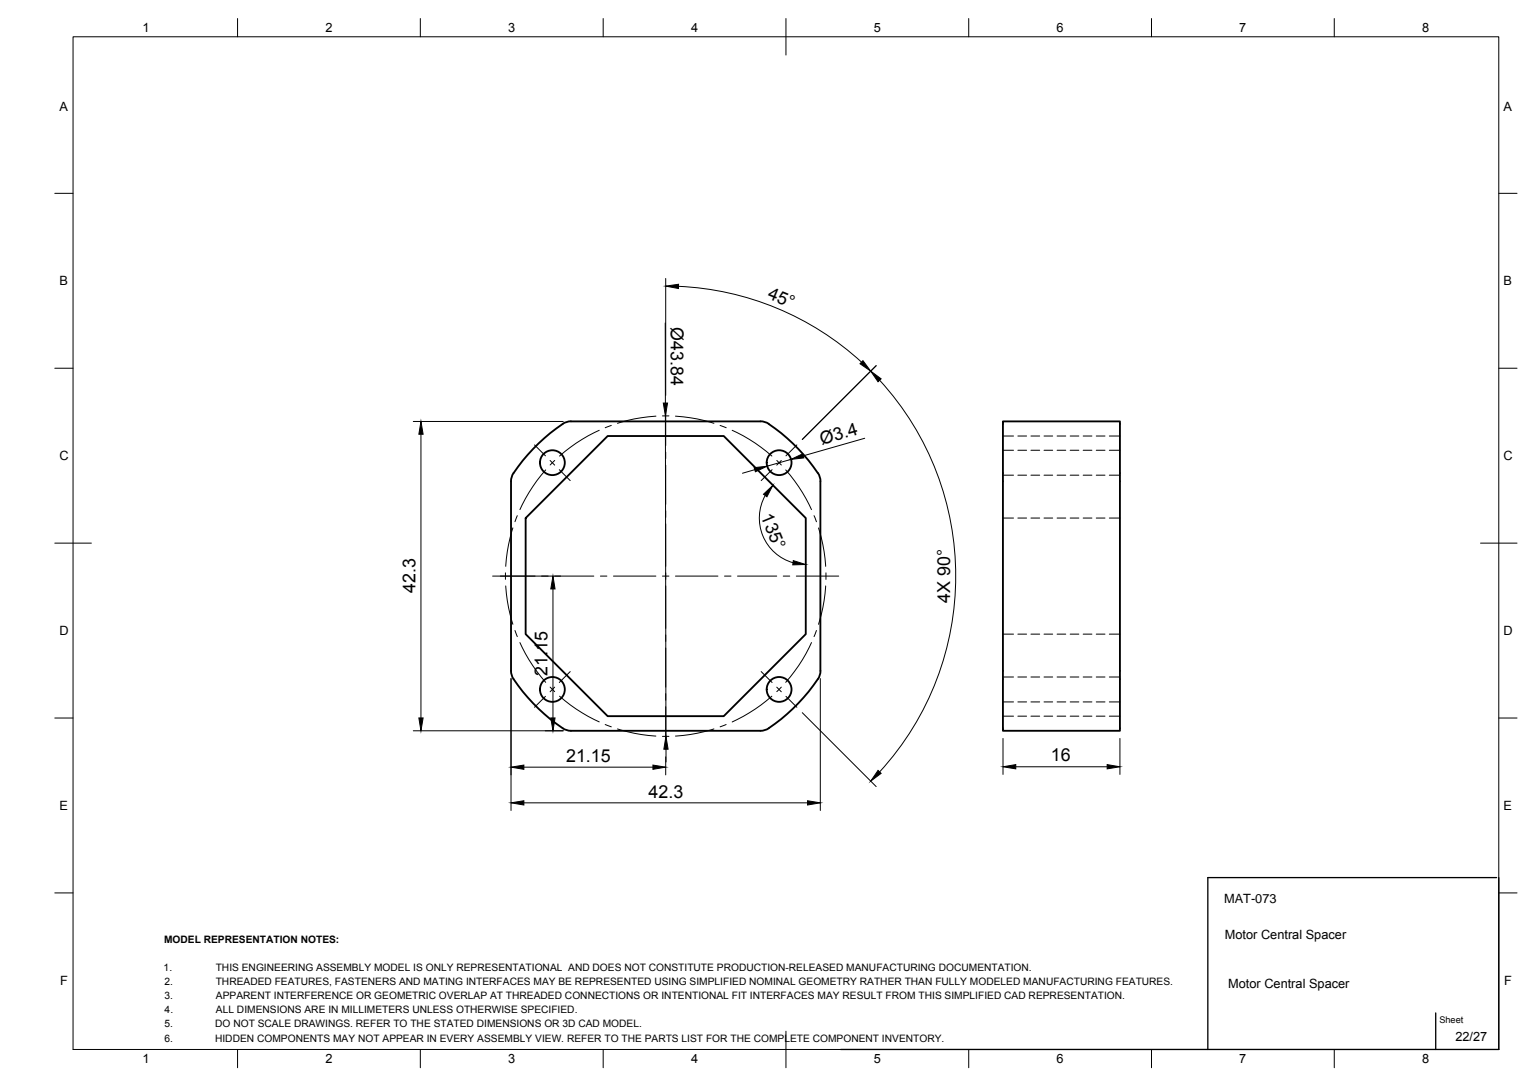
ISO-10303-21;
HEADER;
/* Generated by software containing ST-Developer
 * from STEP Tools, Inc. (www.steptools.com) 
 */

FILE_DESCRIPTION(
/* description */ ('CAx-IF Rec.Pracs.---Representation and Presentation of Product Manufa
cturing Information (PMI)---4.0---2014-10-13'),
/* implementation_level */ '2;1');

FILE_NAME(
/* name */ 'Motor Central Spacer.step',
/* time_stamp */ '2026-10-24T18:52:33-07:00',
/* author */ (''),
/* organization */ (''),
/* preprocessor_version */ 'ST-DEVELOPER v20.2',
/* originating_system */ 'Autodesk Translation Framework v15.17.0.0',
/* authorisation */ '');

FILE_SCHEMA (('AP242_MANAGED_MODEL_BASED_3D_ENGINEERING_MIM_LF { 1 0 10303 442 2 1 4 }'));
ENDSEC;

DATA;
#10=MECHANICAL_DESIGN_GEOMETRIC_PRESENTATION_REPRESENTATION('',(#438),#34876);
#372=SHAPE_REPRESENTATION_RELATIONSHIP('SRR','None',#35009,#405);
#405=ADVANCED_BREP_SHAPE_REPRESENTATION('',(#471),#34867);
#438=STYLED_ITEM('',(#35166),#471);
#471=MANIFOLD_SOLID_BREP('Motor Central Spacer',#19578);
#562=FACE_BOUND('',#6740,.T.);
#563=FACE_BOUND('',#6741,.T.);
#564=FACE_BOUND('',#6742,.T.);
#565=FACE_BOUND('',#6743,.T.);
#566=FACE_BOUND('',#6744,.T.);
#567=FACE_BOUND('',#6759,.T.);
#568=FACE_BOUND('',#6760,.T.);
#569=FACE_BOUND('',#6761,.T.);
#570=FACE_BOUND('',#6762,.T.);
#571=FACE_BOUND('',#6763,.T.);
#951=PLANE('',#21764);
#952=PLANE('',#21774);
#953=PLANE('',#21784);
#954=PLANE('',#21794);
#955=PLANE('',#21798);
#956=PLANE('',#21814);
#957=PLANE('',#21815);
#958=PLANE('',#21816);
#959=PLANE('',#21817);
#960=PLANE('',#21818);
#961=PLANE('',#21819);
#962=PLANE('',#21820);
#963=PLANE('',#21821);
#964=PLANE('',#21822);
#2253=LINE('',#33212,#3852);
#2254=LINE('',#33216,#3853);
#2255=LINE('',#33221,#3854);
#2256=LINE('',#33222,#3855);
#2257=LINE('',#33223,#3856);
#2258=LINE('',#33227,#3857);
#2259=LINE('',#33233,#3858);
#2260=LINE('',#33239,#3859);
#2261=LINE('',#33245,#3860);
#2262=LINE('',#33246,#3861);
#2263=LINE('',#33247,#3862);
#2264=LINE('',#33251,#3863);
#2265=LINE('',#33257,#3864);
#2266=LINE('',#33263,#3865);
#2267=LINE('',#33267,#3866);
#2268=LINE('',#33271,#3867);
#2269=LINE('',#33273,#3868);
#2270=LINE('',#33274,#3869);
#2271=LINE('',#33279,#3870);
#2272=LINE('',#33285,#3871);
#2273=LINE('',#33291,#3872);
#2274=LINE('',#33295,#3873);
#2275=LINE('',#33297,#3874);
#2276=LINE('',#33298,#3875);
#2277=LINE('',#33314,#3876);
#2278=LINE('',#33316,#3877);
#2279=LINE('',#33318,#3878);
#2280=LINE('',#33320,#3879);
#2281=LINE('',#33322,#3880);
#2282=LINE('',#33324,#3881);
#2283=LINE('',#33326,#3882);
#2284=LINE('',#33327,#3883);
#2285=LINE('',#33332,#3884);
#2286=LINE('',#33336,#3885);
#2287=LINE('',#33340,#3886);
#2288=LINE('',#33344,#3887);
#2289=LINE('',#33348,#3888);
#2290=LINE('',#33350,#3889);
#2291=LINE('',#33351,#3890);
#2292=LINE('',#33354,#3891);
#2293=LINE('',#33355,#3892);
#2294=LINE('',#33358,#3893);
#2295=LINE('',#33359,#3894);
#2296=LINE('',#33362,#3895);
#2297=LINE('',#33363,#3896);
#2298=LINE('',#33366,#3897);
#2299=LINE('',#33367,#3898);
#2300=LINE('',#33370,#3899);
#2301=LINE('',#33371,#3900);
#2302=LINE('',#33374,#3901);
#2303=LINE('',#33375,#3902);
#2304=LINE('',#33377,#3903);
#3852=VECTOR('',#27050,0.01);
#3853=VECTOR('',#27053,0.01);
#3854=VECTOR('',#27058,0.01);
#3855=VECTOR('',#27059,1.);
#3856=VECTOR('',#27060,1.);
#3857=VECTOR('',#27063,0.01);
#3858=VECTOR('',#27070,0.01);
#3859=VECTOR('',#27077,0.01);
#3860=VECTOR('',#27084,0.01);
#3861=VECTOR('',#27085,1.);
#3862=VECTOR('',#27086,1.);
#3863=VECTOR('',#27089,1.);
#3864=VECTOR('',#27096,1.);
#3865=VECTOR('',#27103,0.01);
#3866=VECTOR('',#27106,0.01);
#3867=VECTOR('',#27111,1.);
#3868=VECTOR('',#27112,0.01);
#3869=VECTOR('',#27113,1.);
#3870=VECTOR('',#27118,0.01);
#3871=VECTOR('',#27125,0.01);
#3872=VECTOR('',#27132,0.01);
#3873=VECTOR('',#27137,1.);
#3874=VECTOR('',#27138,0.01);
#3875=VECTOR('',#27139,1.);
#3876=VECTOR('',#27158,1.);
#3877=VECTOR('',#27159,1.);
#3878=VECTOR('',#27160,1.);
#3879=VECTOR('',#27161,1.);
#3880=VECTOR('',#27162,1.);
#3881=VECTOR('',#27163,1.);
#3882=VECTOR('',#27164,1.);
#3883=VECTOR('',#27165,1.);
#3884=VECTOR('',#27172,0.0017);
#3885=VECTOR('',#27177,0.0017);
#3886=VECTOR('',#27182,0.0017);
#3887=VECTOR('',#27187,0.0017);
#3888=VECTOR('',#27192,1.);
#3889=VECTOR('',#27193,1.);
#3890=VECTOR('',#27194,1.);
#3891=VECTOR('',#27197,1.);
#3892=VECTOR('',#27198,1.);
#3893=VECTOR('',#27201,1.);
#3894=VECTOR('',#27202,1.);
#3895=VECTOR('',#27205,1.);
#3896=VECTOR('',#27206,1.);
#3897=VECTOR('',#27209,1.);
#3898=VECTOR('',#27210,1.);
#3899=VECTOR('',#27213,1.);
#3900=VECTOR('',#27214,1.);
#3901=VECTOR('',#27217,1.);
#3902=VECTOR('',#27218,1.);
#3903=VECTOR('',#27221,1.);
#4704=CYLINDRICAL_SURFACE('',#21761,0.002);
#4705=CYLINDRICAL_SURFACE('',#21765,0.002);
#4706=CYLINDRICAL_SURFACE('',#21768,0.025125);
#4707=CYLINDRICAL_SURFACE('',#21771,0.002);
#4708=CYLINDRICAL_SURFACE('',#21775,0.002);
#4709=CYLINDRICAL_SURFACE('',#21778,0.025125);
#4710=CYLINDRICAL_SURFACE('',#21781,0.002);
#4711=CYLINDRICAL_SURFACE('',#21785,0.002);
#4712=CYLINDRICAL_SURFACE('',#21788,0.025125);
#4713=CYLINDRICAL_SURFACE('',#21791,0.002);
#4714=CYLINDRICAL_SURFACE('',#21795,0.002);
#4715=CYLINDRICAL_SURFACE('',#21804,0.025125);
#4716=CYLINDRICAL_SURFACE('',#21806,0.0017);
#4717=CYLINDRICAL_SURFACE('',#21808,0.0017);
#4718=CYLINDRICAL_SURFACE('',#21810,0.0017);
#4719=CYLINDRICAL_SURFACE('',#21812,0.0017);
#5597=FACE_OUTER_BOUND('',#6724,.T.);
#5598=FACE_OUTER_BOUND('',#6725,.T.);
#5599=FACE_OUTER_BOUND('',#6726,.T.);
#5600=FACE_OUTER_BOUND('',#6727,.T.);
#5601=FACE_OUTER_BOUND('',#6728,.T.);
#5602=FACE_OUTER_BOUND('',#6729,.T.);
#5603=FACE_OUTER_BOUND('',#6730,.T.);
#5604=FACE_OUTER_BOUND('',#6731,.T.);
#5605=FACE_OUTER_BOUND('',#6732,.T.);
#5606=FACE_OUTER_BOUND('',#6733,.T.);
#5607=FACE_OUTER_BOUND('',#6734,.T.);
#5608=FACE_OUTER_BOUND('',#6735,.T.);
#5609=FACE_OUTER_BOUND('',#6736,.T.);
#5610=FACE_OUTER_BOUND('',#6737,.T.);
#5611=FACE_OUTER_BOUND('',#6738,.T.);
#5612=FACE_OUTER_BOUND('',#6739,.T.);
#5613=FACE_OUTER_BOUND('',#6745,.T.);
#5614=FACE_OUTER_BOUND('',#6746,.T.);
#5615=FACE_OUTER_BOUND('',#6747,.T.);
#5616=FACE_OUTER_BOUND('',#6748,.T.);
#5617=FACE_OUTER_BOUND('',#6749,.T.);
#5618=FACE_OUTER_BOUND('',#6750,.T.);
#5619=FACE_OUTER_BOUND('',#6751,.T.);
#5620=FACE_OUTER_BOUND('',#6752,.T.);
#5621=FACE_OUTER_BOUND('',#6753,.T.);
#5622=FACE_OUTER_BOUND('',#6754,.T.);
#5623=FACE_OUTER_BOUND('',#6755,.T.);
#5624=FACE_OUTER_BOUND('',#6756,.T.);
#5625=FACE_OUTER_BOUND('',#6757,.T.);
#5626=FACE_OUTER_BOUND('',#6758,.T.);
#6724=EDGE_LOOP('',(#17150,#17151,#17152,#17153));
#6725=EDGE_LOOP('',(#17154,#17155,#17156,#17157));
#6726=EDGE_LOOP('',(#17158,#17159,#17160,#17161));
#6727=EDGE_LOOP('',(#17162,#17163,#17164,#17165));
#6728=EDGE_LOOP('',(#17166,#17167,#17168,#17169));
#6729=EDGE_LOOP('',(#17170,#17171,#17172,#17173));
#6730=EDGE_LOOP('',(#17174,#17175,#17176,#17177));
#6731=EDGE_LOOP('',(#17178,#17179,#17180,#17181));
#6732=EDGE_LOOP('',(#17182,#17183,#17184,#17185));
#6733=EDGE_LOOP('',(#17186,#17187,#17188,#17189));
#6734=EDGE_LOOP('',(#17190,#17191,#17192,#17193));
#6735=EDGE_LOOP('',(#17194,#17195,#17196,#17197));
#6736=EDGE_LOOP('',(#17198,#17199,#17200,#17201));
#6737=EDGE_LOOP('',(#17202,#17203,#17204,#17205));
#6738=EDGE_LOOP('',(#17206,#17207,#17208,#17209));
#6739=EDGE_LOOP('',(#17210,#17211,#17212,#17213,#17214,#17215,#17216,#17217,
#17218,#17219,#17220,#17221,#17222,#17223,#17224,#17225));
#6740=EDGE_LOOP('',(#17226));
#6741=EDGE_LOOP('',(#17227));
#6742=EDGE_LOOP('',(#17228));
#6743=EDGE_LOOP('',(#17229));
#6744=EDGE_LOOP('',(#17230,#17231,#17232,#17233,#17234,#17235,#17236,#17237));
#6745=EDGE_LOOP('',(#17238,#17239,#17240,#17241));
#6746=EDGE_LOOP('',(#17242,#17243,#17244,#17245));
#6747=EDGE_LOOP('',(#17246,#17247,#17248,#17249));
#6748=EDGE_LOOP('',(#17250,#17251,#17252,#17253));
#6749=EDGE_LOOP('',(#17254,#17255,#17256,#17257));
#6750=EDGE_LOOP('',(#17258,#17259,#17260,#17261));
#6751=EDGE_LOOP('',(#17262,#17263,#17264,#17265));
#6752=EDGE_LOOP('',(#17266,#17267,#17268,#17269));
#6753=EDGE_LOOP('',(#17270,#17271,#17272,#17273));
#6754=EDGE_LOOP('',(#17274,#17275,#17276,#17277));
#6755=EDGE_LOOP('',(#17278,#17279,#17280,#17281));
#6756=EDGE_LOOP('',(#17282,#17283,#17284,#17285));
#6757=EDGE_LOOP('',(#17286,#17287,#17288,#17289));
#6758=EDGE_LOOP('',(#17290,#17291,#17292,#17293,#17294,#17295,#17296,#17297,
#17298,#17299,#17300,#17301,#17302,#17303,#17304,#17305));
#6759=EDGE_LOOP('',(#17306));
#6760=EDGE_LOOP('',(#17307));
#6761=EDGE_LOOP('',(#17308));
#6762=EDGE_LOOP('',(#17309));
#6763=EDGE_LOOP('',(#17310,#17311,#17312,#17313,#17314,#17315,#17316,#17317));
#7861=CIRCLE('',#21762,0.00200000000001249);
#7862=CIRCLE('',#21763,0.00200000000001249);
#7863=CIRCLE('',#21766,0.00200000000001249);
#7864=CIRCLE('',#21767,0.00200000000001249);
#7865=CIRCLE('',#21769,0.0251250000000138);
#7866=CIRCLE('',#21770,0.0251250000000138);
#7867=CIRCLE('',#21772,0.00200000000001249);
#7868=CIRCLE('',#21773,0.00200000000001249);
#7869=CIRCLE('',#21776,0.00200000000001249);
#7870=CIRCLE('',#21777,0.00200000000001249);
#7871=CIRCLE('',#21779,0.0251250000000138);
#7872=CIRCLE('',#21780,0.0251250000000138);
#7873=CIRCLE('',#21782,0.00200000000001249);
#7874=CIRCLE('',#21783,0.00200000000001249);
#7875=CIRCLE('',#21786,0.00200000000001249);
#7876=CIRCLE('',#21787,0.00200000000001249);
#7877=CIRCLE('',#21789,0.0251250000000138);
#7878=CIRCLE('',#21790,0.0251250000000138);
#7879=CIRCLE('',#21792,0.00200000000001249);
#7880=CIRCLE('',#21793,0.00200000000001249);
#7881=CIRCLE('',#21796,0.00200000000001249);
#7882=CIRCLE('',#21797,0.00200000000001249);
#7883=CIRCLE('',#21799,0.0251250000000138);
#7884=CIRCLE('',#21800,0.00170000000001);
#7885=CIRCLE('',#21801,0.00170000000001);
#7886=CIRCLE('',#21802,0.00170000000001);
#7887=CIRCLE('',#21803,0.00170000000001);
#7888=CIRCLE('',#21805,0.0251250000000138);
#7889=CIRCLE('',#21807,0.00170000000001);
#7890=CIRCLE('',#21809,0.00170000000001);
#7891=CIRCLE('',#21811,0.00170000000001);
#7892=CIRCLE('',#21813,0.00170000000001);
#9513=VERTEX_POINT('',#33210);
#9514=VERTEX_POINT('',#33211);
#9515=VERTEX_POINT('',#33213);
#9516=VERTEX_POINT('',#33215);
#9517=VERTEX_POINT('',#33219);
#9518=VERTEX_POINT('',#33220);
#9519=VERTEX_POINT('',#33225);
#9520=VERTEX_POINT('',#33226);
#9521=VERTEX_POINT('',#33231);
#9522=VERTEX_POINT('',#33232);
#9523=VERTEX_POINT('',#33237);
#9524=VERTEX_POINT('',#33238);
#9525=VERTEX_POINT('',#33243);
#9526=VERTEX_POINT('',#33244);
#9527=VERTEX_POINT('',#33249);
#9528=VERTEX_POINT('',#33250);
#9529=VERTEX_POINT('',#33255);
#9530=VERTEX_POINT('',#33256);
#9531=VERTEX_POINT('',#33261);
#9532=VERTEX_POINT('',#33262);
#9533=VERTEX_POINT('',#33264);
#9534=VERTEX_POINT('',#33266);
#9535=VERTEX_POINT('',#33270);
#9536=VERTEX_POINT('',#33272);
#9537=VERTEX_POINT('',#33276);
#9538=VERTEX_POINT('',#33278);
#9539=VERTEX_POINT('',#33282);
#9540=VERTEX_POINT('',#33284);
#9541=VERTEX_POINT('',#33288);
#9542=VERTEX_POINT('',#33290);
#9543=VERTEX_POINT('',#33294);
#9544=VERTEX_POINT('',#33296);
#9545=VERTEX_POINT('',#33304);
#9546=VERTEX_POINT('',#33306);
#9547=VERTEX_POINT('',#33308);
#9548=VERTEX_POINT('',#33310);
#9549=VERTEX_POINT('',#33312);
#9550=VERTEX_POINT('',#33313);
#9551=VERTEX_POINT('',#33315);
#9552=VERTEX_POINT('',#33317);
#9553=VERTEX_POINT('',#33319);
#9554=VERTEX_POINT('',#33321);
#9555=VERTEX_POINT('',#33323);
#9556=VERTEX_POINT('',#33325);
#9557=VERTEX_POINT('',#33331);
#9558=VERTEX_POINT('',#33335);
#9559=VERTEX_POINT('',#33339);
#9560=VERTEX_POINT('',#33343);
#9561=VERTEX_POINT('',#33347);
#9562=VERTEX_POINT('',#33349);
#9563=VERTEX_POINT('',#33353);
#9564=VERTEX_POINT('',#33357);
#9565=VERTEX_POINT('',#33361);
#9566=VERTEX_POINT('',#33365);
#9567=VERTEX_POINT('',#33369);
#9568=VERTEX_POINT('',#33373);
#12133=EDGE_CURVE('',#9513,#9514,#2253,.T.);
#12134=EDGE_CURVE('',#9514,#9515,#7861,.T.);
#12135=EDGE_CURVE('',#9516,#9515,#2254,.T.);
#12136=EDGE_CURVE('',#9516,#9513,#7862,.T.);
#12137=EDGE_CURVE('',#9517,#9518,#2255,.T.);
#12138=EDGE_CURVE('',#9514,#9518,#2256,.T.);
#12139=EDGE_CURVE('',#9517,#9513,#2257,.T.);
#12140=EDGE_CURVE('',#9519,#9520,#2258,.T.);
#12141=EDGE_CURVE('',#9520,#9518,#7863,.T.);
#12142=EDGE_CURVE('',#9517,#9519,#7864,.T.);
#12143=EDGE_CURVE('',#9521,#9522,#2259,.T.);
#12144=EDGE_CURVE('',#9520,#9522,#7865,.T.);
#12145=EDGE_CURVE('',#9521,#9519,#7866,.T.);
#12146=EDGE_CURVE('',#9523,#9524,#2260,.T.);
#12147=EDGE_CURVE('',#9524,#9522,#7867,.T.);
#12148=EDGE_CURVE('',#9521,#9523,#7868,.T.);
#12149=EDGE_CURVE('',#9525,#9526,#2261,.T.);
#12150=EDGE_CURVE('',#9524,#9526,#2262,.T.);
#12151=EDGE_CURVE('',#9525,#9523,#2263,.T.);
#12152=EDGE_CURVE('',#9527,#9528,#2264,.T.);
#12153=EDGE_CURVE('',#9528,#9526,#7869,.T.);
#12154=EDGE_CURVE('',#9525,#9527,#7870,.T.);
#12155=EDGE_CURVE('',#9529,#9530,#2265,.T.);
#12156=EDGE_CURVE('',#9528,#9529,#7871,.T.);
#12157=EDGE_CURVE('',#9530,#9527,#7872,.T.);
#12158=EDGE_CURVE('',#9531,#9532,#2266,.T.);
#12159=EDGE_CURVE('',#9532,#9533,#7873,.T.);
#12160=EDGE_CURVE('',#9534,#9533,#2267,.T.);
#12161=EDGE_CURVE('',#9534,#9531,#7874,.T.);
#12162=EDGE_CURVE('',#9535,#9533,#2268,.T.);
#12163=EDGE_CURVE('',#9536,#9535,#2269,.T.);
#12164=EDGE_CURVE('',#9534,#9536,#2270,.T.);
#12165=EDGE_CURVE('',#9535,#9537,#7875,.T.);
#12166=EDGE_CURVE('',#9538,#9537,#2271,.T.);
#12167=EDGE_CURVE('',#9538,#9536,#7876,.T.);
#12168=EDGE_CURVE('',#9539,#9537,#7877,.T.);
#12169=EDGE_CURVE('',#9540,#9539,#2272,.T.);
#12170=EDGE_CURVE('',#9538,#9540,#7878,.T.);
#12171=EDGE_CURVE('',#9539,#9541,#7879,.T.);
#12172=EDGE_CURVE('',#9542,#9541,#2273,.T.);
#12173=EDGE_CURVE('',#9542,#9540,#7880,.T.);
#12174=EDGE_CURVE('',#9543,#9541,#2274,.T.);
#12175=EDGE_CURVE('',#9544,#9543,#2275,.T.);
#12176=EDGE_CURVE('',#9542,#9544,#2276,.T.);
#12177=EDGE_CURVE('',#9543,#9529,#7881,.T.);
#12178=EDGE_CURVE('',#9530,#9544,#7882,.T.);
#12179=EDGE_CURVE('',#9532,#9515,#7883,.T.);
#12180=EDGE_CURVE('',#9545,#9545,#7884,.T.);
#12181=EDGE_CURVE('',#9546,#9546,#7885,.T.);
#12182=EDGE_CURVE('',#9547,#9547,#7886,.T.);
#12183=EDGE_CURVE('',#9548,#9548,#7887,.T.);
#12184=EDGE_CURVE('',#9549,#9550,#2277,.T.);
#12185=EDGE_CURVE('',#9550,#9551,#2278,.T.);
#12186=EDGE_CURVE('',#9551,#9552,#2279,.T.);
#12187=EDGE_CURVE('',#9552,#9553,#2280,.T.);
#12188=EDGE_CURVE('',#9553,#9554,#2281,.T.);
#12189=EDGE_CURVE('',#9554,#9555,#2282,.T.);
#12190=EDGE_CURVE('',#9555,#9556,#2283,.T.);
#12191=EDGE_CURVE('',#9556,#9549,#2284,.T.);
#12192=EDGE_CURVE('',#9516,#9531,#7888,.T.);
#12193=EDGE_CURVE('',#9545,#9557,#2285,.T.);
#12194=EDGE_CURVE('',#9557,#9557,#7889,.T.);
#12195=EDGE_CURVE('',#9546,#9558,#2286,.T.);
#12196=EDGE_CURVE('',#9558,#9558,#7890,.T.);
#12197=EDGE_CURVE('',#9547,#9559,#2287,.T.);
#12198=EDGE_CURVE('',#9559,#9559,#7891,.T.);
#12199=EDGE_CURVE('',#9548,#9560,#2288,.T.);
#12200=EDGE_CURVE('',#9560,#9560,#7892,.T.);
#12201=EDGE_CURVE('',#9561,#9550,#2289,.T.);
#12202=EDGE_CURVE('',#9562,#9561,#2290,.T.);
#12203=EDGE_CURVE('',#9551,#9562,#2291,.T.);
#12204=EDGE_CURVE('',#9563,#9562,#2292,.T.);
#12205=EDGE_CURVE('',#9552,#9563,#2293,.T.);
#12206=EDGE_CURVE('',#9564,#9563,#2294,.T.);
#12207=EDGE_CURVE('',#9553,#9564,#2295,.T.);
#12208=EDGE_CURVE('',#9565,#9564,#2296,.T.);
#12209=EDGE_CURVE('',#9554,#9565,#2297,.T.);
#12210=EDGE_CURVE('',#9566,#9565,#2298,.T.);
#12211=EDGE_CURVE('',#9555,#9566,#2299,.T.);
#12212=EDGE_CURVE('',#9567,#9566,#2300,.T.);
#12213=EDGE_CURVE('',#9556,#9567,#2301,.T.);
#12214=EDGE_CURVE('',#9568,#9567,#2302,.T.);
#12215=EDGE_CURVE('',#9549,#9568,#2303,.T.);
#12216=EDGE_CURVE('',#9561,#9568,#2304,.T.);
#17150=ORIENTED_EDGE('',*,*,#12133,.T.);
#17151=ORIENTED_EDGE('',*,*,#12134,.T.);
#17152=ORIENTED_EDGE('',*,*,#12135,.F.);
#17153=ORIENTED_EDGE('',*,*,#12136,.T.);
#17154=ORIENTED_EDGE('',*,*,#12137,.T.);
#17155=ORIENTED_EDGE('',*,*,#12138,.F.);
#17156=ORIENTED_EDGE('',*,*,#12133,.F.);
#17157=ORIENTED_EDGE('',*,*,#12139,.F.);
#17158=ORIENTED_EDGE('',*,*,#12140,.T.);
#17159=ORIENTED_EDGE('',*,*,#12141,.T.);
#17160=ORIENTED_EDGE('',*,*,#12137,.F.);
#17161=ORIENTED_EDGE('',*,*,#12142,.T.);
#17162=ORIENTED_EDGE('',*,*,#12143,.T.);
#17163=ORIENTED_EDGE('',*,*,#12144,.F.);
#17164=ORIENTED_EDGE('',*,*,#12140,.F.);
#17165=ORIENTED_EDGE('',*,*,#12145,.F.);
#17166=ORIENTED_EDGE('',*,*,#12146,.T.);
#17167=ORIENTED_EDGE('',*,*,#12147,.T.);
#17168=ORIENTED_EDGE('',*,*,#12143,.F.);
#17169=ORIENTED_EDGE('',*,*,#12148,.T.);
#17170=ORIENTED_EDGE('',*,*,#12149,.T.);
#17171=ORIENTED_EDGE('',*,*,#12150,.F.);
#17172=ORIENTED_EDGE('',*,*,#12146,.F.);
#17173=ORIENTED_EDGE('',*,*,#12151,.F.);
#17174=ORIENTED_EDGE('',*,*,#12152,.T.);
#17175=ORIENTED_EDGE('',*,*,#12153,.T.);
#17176=ORIENTED_EDGE('',*,*,#12149,.F.);
#17177=ORIENTED_EDGE('',*,*,#12154,.T.);
#17178=ORIENTED_EDGE('',*,*,#12155,.F.);
#17179=ORIENTED_EDGE('',*,*,#12156,.F.);
#17180=ORIENTED_EDGE('',*,*,#12152,.F.);
#17181=ORIENTED_EDGE('',*,*,#12157,.F.);
#17182=ORIENTED_EDGE('',*,*,#12158,.T.);
#17183=ORIENTED_EDGE('',*,*,#12159,.T.);
#17184=ORIENTED_EDGE('',*,*,#12160,.F.);
#17185=ORIENTED_EDGE('',*,*,#12161,.T.);
#17186=ORIENTED_EDGE('',*,*,#12160,.T.);
#17187=ORIENTED_EDGE('',*,*,#12162,.F.);
#17188=ORIENTED_EDGE('',*,*,#12163,.F.);
#17189=ORIENTED_EDGE('',*,*,#12164,.F.);
#17190=ORIENTED_EDGE('',*,*,#12163,.T.);
#17191=ORIENTED_EDGE('',*,*,#12165,.T.);
#17192=ORIENTED_EDGE('',*,*,#12166,.F.);
#17193=ORIENTED_EDGE('',*,*,#12167,.T.);
#17194=ORIENTED_EDGE('',*,*,#12166,.T.);
#17195=ORIENTED_EDGE('',*,*,#12168,.F.);
#17196=ORIENTED_EDGE('',*,*,#12169,.F.);
#17197=ORIENTED_EDGE('',*,*,#12170,.F.);
#17198=ORIENTED_EDGE('',*,*,#12169,.T.);
#17199=ORIENTED_EDGE('',*,*,#12171,.T.);
#17200=ORIENTED_EDGE('',*,*,#12172,.F.);
#17201=ORIENTED_EDGE('',*,*,#12173,.T.);
#17202=ORIENTED_EDGE('',*,*,#12172,.T.);
#17203=ORIENTED_EDGE('',*,*,#12174,.F.);
#17204=ORIENTED_EDGE('',*,*,#12175,.F.);
#17205=ORIENTED_EDGE('',*,*,#12176,.F.);
#17206=ORIENTED_EDGE('',*,*,#12175,.T.);
#17207=ORIENTED_EDGE('',*,*,#12177,.T.);
#17208=ORIENTED_EDGE('',*,*,#12155,.T.);
#17209=ORIENTED_EDGE('',*,*,#12178,.T.);
#17210=ORIENTED_EDGE('',*,*,#12159,.F.);
#17211=ORIENTED_EDGE('',*,*,#12179,.T.);
#17212=ORIENTED_EDGE('',*,*,#12134,.F.);
#17213=ORIENTED_EDGE('',*,*,#12138,.T.);
#17214=ORIENTED_EDGE('',*,*,#12141,.F.);
#17215=ORIENTED_EDGE('',*,*,#12144,.T.);
#17216=ORIENTED_EDGE('',*,*,#12147,.F.);
#17217=ORIENTED_EDGE('',*,*,#12150,.T.);
#17218=ORIENTED_EDGE('',*,*,#12153,.F.);
#17219=ORIENTED_EDGE('',*,*,#12156,.T.);
#17220=ORIENTED_EDGE('',*,*,#12177,.F.);
#17221=ORIENTED_EDGE('',*,*,#12174,.T.);
#17222=ORIENTED_EDGE('',*,*,#12171,.F.);
#17223=ORIENTED_EDGE('',*,*,#12168,.T.);
#17224=ORIENTED_EDGE('',*,*,#12165,.F.);
#17225=ORIENTED_EDGE('',*,*,#12162,.T.);
#17226=ORIENTED_EDGE('',*,*,#12180,.T.);
#17227=ORIENTED_EDGE('',*,*,#12181,.T.);
#17228=ORIENTED_EDGE('',*,*,#12182,.T.);
#17229=ORIENTED_EDGE('',*,*,#12183,.T.);
#17230=ORIENTED_EDGE('',*,*,#12184,.T.);
#17231=ORIENTED_EDGE('',*,*,#12185,.T.);
#17232=ORIENTED_EDGE('',*,*,#12186,.T.);
#17233=ORIENTED_EDGE('',*,*,#12187,.T.);
#17234=ORIENTED_EDGE('',*,*,#12188,.T.);
#17235=ORIENTED_EDGE('',*,*,#12189,.T.);
#17236=ORIENTED_EDGE('',*,*,#12190,.T.);
#17237=ORIENTED_EDGE('',*,*,#12191,.T.);
#17238=ORIENTED_EDGE('',*,*,#12135,.T.);
#17239=ORIENTED_EDGE('',*,*,#12179,.F.);
#17240=ORIENTED_EDGE('',*,*,#12158,.F.);
#17241=ORIENTED_EDGE('',*,*,#12192,.F.);
#17242=ORIENTED_EDGE('',*,*,#12180,.F.);
#17243=ORIENTED_EDGE('',*,*,#12193,.T.);
#17244=ORIENTED_EDGE('',*,*,#12194,.F.);
#17245=ORIENTED_EDGE('',*,*,#12193,.F.);
#17246=ORIENTED_EDGE('',*,*,#12181,.F.);
#17247=ORIENTED_EDGE('',*,*,#12195,.T.);
#17248=ORIENTED_EDGE('',*,*,#12196,.F.);
#17249=ORIENTED_EDGE('',*,*,#12195,.F.);
#17250=ORIENTED_EDGE('',*,*,#12182,.F.);
#17251=ORIENTED_EDGE('',*,*,#12197,.T.);
#17252=ORIENTED_EDGE('',*,*,#12198,.F.);
#17253=ORIENTED_EDGE('',*,*,#12197,.F.);
#17254=ORIENTED_EDGE('',*,*,#12183,.F.);
#17255=ORIENTED_EDGE('',*,*,#12199,.T.);
#17256=ORIENTED_EDGE('',*,*,#12200,.F.);
#17257=ORIENTED_EDGE('',*,*,#12199,.F.);
#17258=ORIENTED_EDGE('',*,*,#12201,.F.);
#17259=ORIENTED_EDGE('',*,*,#12202,.F.);
#17260=ORIENTED_EDGE('',*,*,#12203,.F.);
#17261=ORIENTED_EDGE('',*,*,#12185,.F.);
#17262=ORIENTED_EDGE('',*,*,#12203,.T.);
#17263=ORIENTED_EDGE('',*,*,#12204,.F.);
#17264=ORIENTED_EDGE('',*,*,#12205,.F.);
#17265=ORIENTED_EDGE('',*,*,#12186,.F.);
#17266=ORIENTED_EDGE('',*,*,#12205,.T.);
#17267=ORIENTED_EDGE('',*,*,#12206,.F.);
#17268=ORIENTED_EDGE('',*,*,#12207,.F.);
#17269=ORIENTED_EDGE('',*,*,#12187,.F.);
#17270=ORIENTED_EDGE('',*,*,#12207,.T.);
#17271=ORIENTED_EDGE('',*,*,#12208,.F.);
#17272=ORIENTED_EDGE('',*,*,#12209,.F.);
#17273=ORIENTED_EDGE('',*,*,#12188,.F.);
#17274=ORIENTED_EDGE('',*,*,#12209,.T.);
#17275=ORIENTED_EDGE('',*,*,#12210,.F.);
#17276=ORIENTED_EDGE('',*,*,#12211,.F.);
#17277=ORIENTED_EDGE('',*,*,#12189,.F.);
#17278=ORIENTED_EDGE('',*,*,#12211,.T.);
#17279=ORIENTED_EDGE('',*,*,#12212,.F.);
#17280=ORIENTED_EDGE('',*,*,#12213,.F.);
#17281=ORIENTED_EDGE('',*,*,#12190,.F.);
#17282=ORIENTED_EDGE('',*,*,#12213,.T.);
#17283=ORIENTED_EDGE('',*,*,#12214,.F.);
#17284=ORIENTED_EDGE('',*,*,#12215,.F.);
#17285=ORIENTED_EDGE('',*,*,#12191,.F.);
#17286=ORIENTED_EDGE('',*,*,#12215,.T.);
#17287=ORIENTED_EDGE('',*,*,#12216,.F.);
#17288=ORIENTED_EDGE('',*,*,#12201,.T.);
#17289=ORIENTED_EDGE('',*,*,#12184,.F.);
#17290=ORIENTED_EDGE('',*,*,#12161,.F.);
#17291=ORIENTED_EDGE('',*,*,#12164,.T.);
#17292=ORIENTED_EDGE('',*,*,#12167,.F.);
#17293=ORIENTED_EDGE('',*,*,#12170,.T.);
#17294=ORIENTED_EDGE('',*,*,#12173,.F.);
#17295=ORIENTED_EDGE('',*,*,#12176,.T.);
#17296=ORIENTED_EDGE('',*,*,#12178,.F.);
#17297=ORIENTED_EDGE('',*,*,#12157,.T.);
#17298=ORIENTED_EDGE('',*,*,#12154,.F.);
#17299=ORIENTED_EDGE('',*,*,#12151,.T.);
#17300=ORIENTED_EDGE('',*,*,#12148,.F.);
#17301=ORIENTED_EDGE('',*,*,#12145,.T.);
#17302=ORIENTED_EDGE('',*,*,#12142,.F.);
#17303=ORIENTED_EDGE('',*,*,#12139,.T.);
#17304=ORIENTED_EDGE('',*,*,#12136,.F.);
#17305=ORIENTED_EDGE('',*,*,#12192,.T.);
#17306=ORIENTED_EDGE('',*,*,#12194,.T.);
#17307=ORIENTED_EDGE('',*,*,#12196,.T.);
#17308=ORIENTED_EDGE('',*,*,#12198,.T.);
#17309=ORIENTED_EDGE('',*,*,#12200,.T.);
#17310=ORIENTED_EDGE('',*,*,#12216,.T.);
#17311=ORIENTED_EDGE('',*,*,#12214,.T.);
#17312=ORIENTED_EDGE('',*,*,#12212,.T.);
#17313=ORIENTED_EDGE('',*,*,#12210,.T.);
#17314=ORIENTED_EDGE('',*,*,#12208,.T.);
#17315=ORIENTED_EDGE('',*,*,#12206,.T.);
#17316=ORIENTED_EDGE('',*,*,#12204,.T.);
#17317=ORIENTED_EDGE('',*,*,#12202,.T.);
#19313=ADVANCED_FACE('',(#5597),#4704,.T.);
#19314=ADVANCED_FACE('',(#5598),#951,.T.);
#19315=ADVANCED_FACE('',(#5599),#4705,.T.);
#19316=ADVANCED_FACE('',(#5600),#4706,.T.);
#19317=ADVANCED_FACE('',(#5601),#4707,.T.);
#19318=ADVANCED_FACE('',(#5602),#952,.T.);
#19319=ADVANCED_FACE('',(#5603),#4708,.T.);
#19320=ADVANCED_FACE('',(#5604),#4709,.T.);
#19321=ADVANCED_FACE('',(#5605),#4710,.T.);
#19322=ADVANCED_FACE('',(#5606),#953,.T.);
#19323=ADVANCED_FACE('',(#5607),#4711,.T.);
#19324=ADVANCED_FACE('',(#5608),#4712,.T.);
#19325=ADVANCED_FACE('',(#5609),#4713,.T.);
#19326=ADVANCED_FACE('',(#5610),#954,.T.);
#19327=ADVANCED_FACE('',(#5611),#4714,.T.);
#19328=ADVANCED_FACE('',(#5612,#562,#563,#564,#565,#566),#955,.F.);
#19329=ADVANCED_FACE('',(#5613),#4715,.T.);
#19330=ADVANCED_FACE('',(#5614),#4716,.F.);
#19331=ADVANCED_FACE('',(#5615),#4717,.F.);
#19332=ADVANCED_FACE('',(#5616),#4718,.F.);
#19333=ADVANCED_FACE('',(#5617),#4719,.F.);
#19334=ADVANCED_FACE('',(#5618),#956,.T.);
#19335=ADVANCED_FACE('',(#5619),#957,.T.);
#19336=ADVANCED_FACE('',(#5620),#958,.T.);
#19337=ADVANCED_FACE('',(#5621),#959,.T.);
#19338=ADVANCED_FACE('',(#5622),#960,.T.);
#19339=ADVANCED_FACE('',(#5623),#961,.T.);
#19340=ADVANCED_FACE('',(#5624),#962,.T.);
#19341=ADVANCED_FACE('',(#5625),#963,.T.);
#19342=ADVANCED_FACE('',(#5626,#567,#568,#569,#570,#571),#964,.T.);
#19578=CLOSED_SHELL('',(#19313,#19314,#19315,#19316,#19317,#19318,#19319,
#19320,#19321,#19322,#19323,#19324,#19325,#19326,#19327,#19328,#19329,#19330,
#19331,#19332,#19333,#19334,#19335,#19336,#19337,#19338,#19339,#19340,#19341,
#19342));
#21760=AXIS2_PLACEMENT_3D('',#33208,#27046,#27047);
#21761=AXIS2_PLACEMENT_3D('',#33209,#27048,#27049);
#21762=AXIS2_PLACEMENT_3D('',#33214,#27051,#27052);
#21763=AXIS2_PLACEMENT_3D('',#33217,#27054,#27055);
#21764=AXIS2_PLACEMENT_3D('',#33218,#27056,#27057);
#21765=AXIS2_PLACEMENT_3D('',#33224,#27061,#27062);
#21766=AXIS2_PLACEMENT_3D('',#33228,#27064,#27065);
#21767=AXIS2_PLACEMENT_3D('',#33229,#27066,#27067);
#21768=AXIS2_PLACEMENT_3D('',#33230,#27068,#27069);
#21769=AXIS2_PLACEMENT_3D('',#33234,#27071,#27072);
#21770=AXIS2_PLACEMENT_3D('',#33235,#27073,#27074);
#21771=AXIS2_PLACEMENT_3D('',#33236,#27075,#27076);
#21772=AXIS2_PLACEMENT_3D('',#33240,#27078,#27079);
#21773=AXIS2_PLACEMENT_3D('',#33241,#27080,#27081);
#21774=AXIS2_PLACEMENT_3D('',#33242,#27082,#27083);
#21775=AXIS2_PLACEMENT_3D('',#33248,#27087,#27088);
#21776=AXIS2_PLACEMENT_3D('',#33252,#27090,#27091);
#21777=AXIS2_PLACEMENT_3D('',#33253,#27092,#27093);
#21778=AXIS2_PLACEMENT_3D('',#33254,#27094,#27095);
#21779=AXIS2_PLACEMENT_3D('',#33258,#27097,#27098);
#21780=AXIS2_PLACEMENT_3D('',#33259,#27099,#27100);
#21781=AXIS2_PLACEMENT_3D('',#33260,#27101,#27102);
#21782=AXIS2_PLACEMENT_3D('',#33265,#27104,#27105);
#21783=AXIS2_PLACEMENT_3D('',#33268,#27107,#27108);
#21784=AXIS2_PLACEMENT_3D('',#33269,#27109,#27110);
#21785=AXIS2_PLACEMENT_3D('',#33275,#27114,#27115);
#21786=AXIS2_PLACEMENT_3D('',#33277,#27116,#27117);
#21787=AXIS2_PLACEMENT_3D('',#33280,#27119,#27120);
#21788=AXIS2_PLACEMENT_3D('',#33281,#27121,#27122);
#21789=AXIS2_PLACEMENT_3D('',#33283,#27123,#27124);
#21790=AXIS2_PLACEMENT_3D('',#33286,#27126,#27127);
#21791=AXIS2_PLACEMENT_3D('',#33287,#27128,#27129);
#21792=AXIS2_PLACEMENT_3D('',#33289,#27130,#27131);
#21793=AXIS2_PLACEMENT_3D('',#33292,#27133,#27134);
#21794=AXIS2_PLACEMENT_3D('',#33293,#27135,#27136);
#21795=AXIS2_PLACEMENT_3D('',#33299,#27140,#27141);
#21796=AXIS2_PLACEMENT_3D('',#33300,#27142,#27143);
#21797=AXIS2_PLACEMENT_3D('',#33301,#27144,#27145);
#21798=AXIS2_PLACEMENT_3D('',#33302,#27146,#27147);
#21799=AXIS2_PLACEMENT_3D('',#33303,#27148,#27149);
#21800=AXIS2_PLACEMENT_3D('',#33305,#27150,#27151);
#21801=AXIS2_PLACEMENT_3D('',#33307,#27152,#27153);
#21802=AXIS2_PLACEMENT_3D('',#33309,#27154,#27155);
#21803=AXIS2_PLACEMENT_3D('',#33311,#27156,#27157);
#21804=AXIS2_PLACEMENT_3D('',#33328,#27166,#27167);
#21805=AXIS2_PLACEMENT_3D('',#33329,#27168,#27169);
#21806=AXIS2_PLACEMENT_3D('',#33330,#27170,#27171);
#21807=AXIS2_PLACEMENT_3D('',#33333,#27173,#27174);
#21808=AXIS2_PLACEMENT_3D('',#33334,#27175,#27176);
#21809=AXIS2_PLACEMENT_3D('',#33337,#27178,#27179);
#21810=AXIS2_PLACEMENT_3D('',#33338,#27180,#27181);
#21811=AXIS2_PLACEMENT_3D('',#33341,#27183,#27184);
#21812=AXIS2_PLACEMENT_3D('',#33342,#27185,#27186);
#21813=AXIS2_PLACEMENT_3D('',#33345,#27188,#27189);
#21814=AXIS2_PLACEMENT_3D('',#33346,#27190,#27191);
#21815=AXIS2_PLACEMENT_3D('',#33352,#27195,#27196);
#21816=AXIS2_PLACEMENT_3D('',#33356,#27199,#27200);
#21817=AXIS2_PLACEMENT_3D('',#33360,#27203,#27204);
#21818=AXIS2_PLACEMENT_3D('',#33364,#27207,#27208);
#21819=AXIS2_PLACEMENT_3D('',#33368,#27211,#27212);
#21820=AXIS2_PLACEMENT_3D('',#33372,#27215,#27216);
#21821=AXIS2_PLACEMENT_3D('',#33376,#27219,#27220);
#21822=AXIS2_PLACEMENT_3D('',#33378,#27222,#27223);
#27046=DIRECTION('axis',(0.,0.,1.));
#27047=DIRECTION('refdir',(1.,0.,0.));
#27048=DIRECTION('center_axis',(0.,1.,0.));
#27049=DIRECTION('ref_axis',(-0.293165390088848,0.,-0.956061741758373));
#27050=DIRECTION('',(0.,-1.,0.));
#27051=DIRECTION('center_axis',(0.,1.,0.));
#27052=DIRECTION('ref_axis',(-0.293165390092017,0.,-0.956061741757401));
#27053=DIRECTION('',(0.,-1.,0.));
#27054=DIRECTION('center_axis',(0.,-1.,0.));
#27055=DIRECTION('ref_axis',(-0.293165390092017,0.,-0.956061741757401));
#27056=DIRECTION('center_axis',(0.,0.,-1.));
#27057=DIRECTION('ref_axis',(0.,-1.,0.));
#27058=DIRECTION('',(0.,-1.,0.));
#27059=DIRECTION('',(1.,0.,0.));
#27060=DIRECTION('',(-1.,0.,0.));
#27061=DIRECTION('center_axis',(0.,1.,0.));
#27062=DIRECTION('ref_axis',(0.293165390088847,0.,-0.956061741758373));
#27063=DIRECTION('',(0.,-1.,0.));
#27064=DIRECTION('center_axis',(0.,1.,0.));
#27065=DIRECTION('ref_axis',(0.293165390092016,0.,-0.956061741757401));
#27066=DIRECTION('center_axis',(0.,-1.,0.));
#27067=DIRECTION('ref_axis',(0.293165390092016,0.,-0.956061741757401));
#27068=DIRECTION('center_axis',(0.,1.,0.));
#27069=DIRECTION('ref_axis',(0.841791044776119,0.,-0.539803516971434));
#27070=DIRECTION('',(0.,-1.,0.));
#27071=DIRECTION('center_axis',(0.,-1.,0.));
#27072=DIRECTION('ref_axis',(0.841791044776055,0.,-0.539803516971535));
#27073=DIRECTION('center_axis',(0.,1.,0.));
#27074=DIRECTION('ref_axis',(0.841791044776055,0.,-0.539803516971535));
#27075=DIRECTION('center_axis',(0.,1.,0.));
#27076=DIRECTION('ref_axis',(0.956061741758373,0.,-0.293165390088847));
#27077=DIRECTION('',(0.,-1.,0.));
#27078=DIRECTION('center_axis',(0.,1.,0.));
#27079=DIRECTION('ref_axis',(0.956061741757401,0.,-0.293165390092016));
#27080=DIRECTION('center_axis',(0.,-1.,0.));
#27081=DIRECTION('ref_axis',(0.956061741757401,0.,-0.293165390092016));
#27082=DIRECTION('center_axis',(1.,2.68038322042824E-32,4.38829015768159E-48));
#27083=DIRECTION('ref_axis',(3.64629801437176E-63,-1.63718759475762E-16,
1.));
#27084=DIRECTION('',(0.,-1.,0.));
#27085=DIRECTION('',(-1.00016371875848E-12,0.,1.));
#27086=DIRECTION('',(1.00016371875848E-12,0.,-1.));
#27087=DIRECTION('center_axis',(0.,1.,0.));
#27088=DIRECTION('ref_axis',(0.956061741758373,0.,0.293165390088847));
#27089=DIRECTION('',(0.,-1.,0.));
#27090=DIRECTION('center_axis',(0.,1.,0.));
#27091=DIRECTION('ref_axis',(0.956061741757401,0.,0.293165390092016));
#27092=DIRECTION('center_axis',(0.,-1.,0.));
#27093=DIRECTION('ref_axis',(0.956061741757401,0.,0.293165390092016));
#27094=DIRECTION('center_axis',(0.,1.,0.));
#27095=DIRECTION('ref_axis',(0.539803516971435,0.,0.841791044776119));
#27096=DIRECTION('',(0.,1.,0.));
#27097=DIRECTION('center_axis',(0.,-1.,0.));
#27098=DIRECTION('ref_axis',(0.539803516971536,0.,0.841791044776054));
#27099=DIRECTION('center_axis',(0.,1.,0.));
#27100=DIRECTION('ref_axis',(0.539803516971536,0.,0.841791044776054));
#27101=DIRECTION('center_axis',(0.,1.,0.));
#27102=DIRECTION('ref_axis',(-0.956061741758373,0.,-0.293165390088847));
#27103=DIRECTION('',(0.,-1.,0.));
#27104=DIRECTION('center_axis',(0.,1.,0.));
#27105=DIRECTION('ref_axis',(-0.956061741757401,0.,-0.293165390092016));
#27106=DIRECTION('',(0.,-1.,0.));
#27107=DIRECTION('center_axis',(0.,-1.,0.));
#27108=DIRECTION('ref_axis',(-0.956061741757401,0.,-0.293165390092016));
#27109=DIRECTION('center_axis',(-1.,0.,0.));
#27110=DIRECTION('ref_axis',(0.,0.,1.));
#27111=DIRECTION('',(0.,0.,-1.));
#27112=DIRECTION('',(0.,-1.,0.));
#27113=DIRECTION('',(0.,0.,1.));
#27114=DIRECTION('center_axis',(0.,-1.,0.));
#27115=DIRECTION('ref_axis',(-0.956061741758373,0.,0.293165390088847));
#27116=DIRECTION('center_axis',(0.,1.,0.));
#27117=DIRECTION('ref_axis',(-0.956061741757401,0.,0.293165390092016));
#27118=DIRECTION('',(0.,-1.,0.));
#27119=DIRECTION('center_axis',(0.,-1.,0.));
#27120=DIRECTION('ref_axis',(-0.956061741757401,0.,0.293165390092016));
#27121=DIRECTION('center_axis',(0.,1.,0.));
#27122=DIRECTION('ref_axis',(-0.841791044776119,0.,0.539803516971435));
#27123=DIRECTION('center_axis',(0.,-1.,0.));
#27124=DIRECTION('ref_axis',(-0.841791044776054,0.,0.539803516971536));
#27125=DIRECTION('',(0.,-1.,0.));
#27126=DIRECTION('center_axis',(0.,1.,0.));
#27127=DIRECTION('ref_axis',(-0.841791044776054,0.,0.539803516971536));
#27128=DIRECTION('center_axis',(0.,1.,0.));
#27129=DIRECTION('ref_axis',(-0.293165390088847,0.,0.956061741758373));
#27130=DIRECTION('center_axis',(0.,1.,0.));
#27131=DIRECTION('ref_axis',(-0.293165390092016,0.,0.956061741757401));
#27132=DIRECTION('',(0.,-1.,0.));
#27133=DIRECTION('center_axis',(0.,-1.,0.));
#27134=DIRECTION('ref_axis',(-0.293165390092016,0.,0.956061741757401));
#27135=DIRECTION('center_axis',(0.,0.,1.));
#27136=DIRECTION('ref_axis',(1.,0.,0.));
#27137=DIRECTION('',(-1.,0.,0.));
#27138=DIRECTION('',(0.,-1.,0.));
#27139=DIRECTION('',(1.,0.,0.));
#27140=DIRECTION('center_axis',(0.,1.,0.));
#27141=DIRECTION('ref_axis',(0.293165390088847,0.,0.956061741758373));
#27142=DIRECTION('center_axis',(0.,1.,0.));
#27143=DIRECTION('ref_axis',(0.293165390092016,0.,0.956061741757401));
#27144=DIRECTION('center_axis',(0.,-1.,0.));
#27145=DIRECTION('ref_axis',(0.293165390092016,0.,0.956061741757401));
#27146=DIRECTION('center_axis',(0.,1.,0.));
#27147=DIRECTION('ref_axis',(1.,0.,0.));
#27148=DIRECTION('center_axis',(0.,-1.,0.));
#27149=DIRECTION('ref_axis',(-0.539803516971535,0.,-0.841791044776055));
#27150=DIRECTION('center_axis',(0.,1.,0.));
#27151=DIRECTION('ref_axis',(1.,0.,0.));
#27152=DIRECTION('center_axis',(0.,1.,0.));
#27153=DIRECTION('ref_axis',(1.,0.,0.));
#27154=DIRECTION('center_axis',(0.,1.,0.));
#27155=DIRECTION('ref_axis',(1.,0.,0.));
#27156=DIRECTION('center_axis',(0.,1.,0.));
#27157=DIRECTION('ref_axis',(1.,0.,0.));
#27158=DIRECTION('',(0.707106781186548,0.,0.707106781186547));
#27159=DIRECTION('',(1.,0.,-1.00027992850901E-12));
#27160=DIRECTION('',(0.707106781186547,0.,-0.707106781186548));
#27161=DIRECTION('',(-1.000139964254E-12,0.,-1.));
#27162=DIRECTION('',(-0.707106781186548,0.,-0.707106781186547));
#27163=DIRECTION('',(-1.,0.,1.000139964254E-12));
#27164=DIRECTION('',(-0.707106781186547,0.,0.707106781186548));
#27165=DIRECTION('',(1.000139964254E-12,0.,1.));
#27166=DIRECTION('center_axis',(0.,1.,0.));
#27167=DIRECTION('ref_axis',(-0.539803516971434,0.,-0.841791044776119));
#27168=DIRECTION('center_axis',(0.,1.,0.));
#27169=DIRECTION('ref_axis',(-0.539803516971535,0.,-0.841791044776055));
#27170=DIRECTION('center_axis',(0.,1.,0.));
#27171=DIRECTION('ref_axis',(1.,0.,0.));
#27172=DIRECTION('',(0.,1.,0.));
#27173=DIRECTION('center_axis',(0.,-1.,0.));
#27174=DIRECTION('ref_axis',(1.,0.,0.));
#27175=DIRECTION('center_axis',(0.,1.,0.));
#27176=DIRECTION('ref_axis',(1.,0.,0.));
#27177=DIRECTION('',(0.,1.,0.));
#27178=DIRECTION('center_axis',(0.,-1.,0.));
#27179=DIRECTION('ref_axis',(1.,0.,0.));
#27180=DIRECTION('center_axis',(0.,1.,0.));
#27181=DIRECTION('ref_axis',(1.,0.,0.));
#27182=DIRECTION('',(0.,1.,0.));
#27183=DIRECTION('center_axis',(0.,-1.,0.));
#27184=DIRECTION('ref_axis',(1.,0.,0.));
#27185=DIRECTION('center_axis',(0.,1.,0.));
#27186=DIRECTION('ref_axis',(1.,0.,0.));
#27187=DIRECTION('',(0.,1.,0.));
#27188=DIRECTION('center_axis',(0.,-1.,0.));
#27189=DIRECTION('ref_axis',(1.,0.,0.));
#27190=DIRECTION('center_axis',(-2.79928510006155E-16,0.,-1.));
#27191=DIRECTION('ref_axis',(-1.,0.,2.79928510006155E-16));
#27192=DIRECTION('',(0.,-1.,0.));
#27193=DIRECTION('',(-1.,0.,1.00027992850901E-12));
#27194=DIRECTION('',(0.,1.,0.));
#27195=DIRECTION('center_axis',(-0.707106781186548,0.,-0.707106781186547));
#27196=DIRECTION('ref_axis',(-0.707106781186547,0.,0.707106781186548));
#27197=DIRECTION('',(-0.707106781186547,0.,0.707106781186548));
#27198=DIRECTION('',(0.,1.,0.));
#27199=DIRECTION('center_axis',(-1.,0.,1.39964255003077E-16));
#27200=DIRECTION('ref_axis',(0.,1.,0.));
#27201=DIRECTION('',(1.000139964254E-12,0.,1.));
#27202=DIRECTION('',(0.,1.,0.));
#27203=DIRECTION('center_axis',(-0.707106781186547,0.,0.707106781186548));
#27204=DIRECTION('ref_axis',(0.,1.,0.));
#27205=DIRECTION('',(0.707106781186548,0.,0.707106781186547));
#27206=DIRECTION('',(0.,1.,0.));
#27207=DIRECTION('center_axis',(2.74189873077128E-48,1.95899926785664E-32,
1.));
#27208=DIRECTION('ref_axis',(1.,-1.39964255003077E-16,-7.02611785152007E-64));
#27209=DIRECTION('',(1.,0.,-1.000139964254E-12));
#27210=DIRECTION('',(0.,1.,0.));
#27211=DIRECTION('center_axis',(0.707106781186548,0.,0.707106781186547));
#27212=DIRECTION('ref_axis',(0.,-1.,0.));
#27213=DIRECTION('',(0.707106781186547,0.,-0.707106781186548));
#27214=DIRECTION('',(0.,1.,0.));
#27215=DIRECTION('center_axis',(1.,0.,-1.39964255003077E-16));
#27216=DIRECTION('ref_axis',(0.,1.,0.));
#27217=DIRECTION('',(-1.000139964254E-12,0.,-1.));
#27218=DIRECTION('',(0.,1.,0.));
#27219=DIRECTION('center_axis',(0.707106781186547,0.,-0.707106781186548));
#27220=DIRECTION('ref_axis',(0.,-1.,0.));
#27221=DIRECTION('',(-0.707106781186548,0.,-0.707106781186547));
#27222=DIRECTION('center_axis',(0.,1.,0.));
#27223=DIRECTION('ref_axis',(1.,0.,0.));
#33208=CARTESIAN_POINT('',(0.,0.,0.));
#33209=CARTESIAN_POINT('Origin',(-0.0129631448730622,-0.016,-0.01915));
#33210=CARTESIAN_POINT('',(-0.0129631448730622,-0.008,-0.02115));
#33211=CARTESIAN_POINT('',(-0.0129631448730622,-0.024,-0.02115));
#33212=CARTESIAN_POINT('',(-0.0129631448730622,-0.008,-0.02115));
#33213=CARTESIAN_POINT('',(-0.0140842817269487,-0.024,-0.0208062162162162));
#33214=CARTESIAN_POINT('Origin',(-0.0129631448730722,-0.02400000000001,
-0.0191500000000101));
#33215=CARTESIAN_POINT('',(-0.0140842817269487,-0.008,-0.0208062162162162));
#33216=CARTESIAN_POINT('',(-0.0140842817269635,-0.008,-0.0208062162162381));
#33217=CARTESIAN_POINT('Origin',(-0.0129631448730722,-0.00799999999999,
-0.0191500000000101));
#33218=CARTESIAN_POINT('Origin',(0.0135625633639073,-0.016,-0.02115));
#33219=CARTESIAN_POINT('',(0.0129631448730622,-0.008,-0.02115));
#33220=CARTESIAN_POINT('',(0.0129631448730622,-0.024,-0.02115));
#33221=CARTESIAN_POINT('',(0.0129631448730622,-0.008,-0.0211500000000226));
#33222=CARTESIAN_POINT('',(0.0135625633639173,-0.02400000000001,-0.02115000000001));
#33223=CARTESIAN_POINT('',(0.0135625633639173,-0.00799999999999,-0.02115000000001));
#33224=CARTESIAN_POINT('Origin',(0.0129631448730622,-0.016,-0.01915));
#33225=CARTESIAN_POINT('',(0.0140842817269487,-0.008,-0.0208062162162162));
#33226=CARTESIAN_POINT('',(0.0140842817269487,-0.024,-0.0208062162162162));
#33227=CARTESIAN_POINT('',(0.0140842817269487,-0.008,-0.0208062162162162));
#33228=CARTESIAN_POINT('Origin',(0.0129631448730722,-0.02400000000001,-0.0191500000000101));
#33229=CARTESIAN_POINT('Origin',(0.0129631448730722,-0.00799999999999,-0.0191500000000101));
#33230=CARTESIAN_POINT('Origin',(-2.55351295663785E-17,-0.016,-3.88578058618804E-17));
#33231=CARTESIAN_POINT('',(0.0208062162162162,-0.008,-0.0140842817269487));
#33232=CARTESIAN_POINT('',(0.0208062162162162,-0.024,-0.0140842817269487));
#33233=CARTESIAN_POINT('',(0.020806216216238,-0.008,-0.0140842817269635));
#33234=CARTESIAN_POINT('Origin',(-1.00255351295664E-14,-0.02400000000001,
9.96114219413812E-15));
#33235=CARTESIAN_POINT('Origin',(-1.00255351295664E-14,-0.00799999999999,
9.96114219413812E-15));
#33236=CARTESIAN_POINT('Origin',(0.01915,-0.016,-0.0129631448730622));
#33237=CARTESIAN_POINT('',(0.02115,-0.008,-0.0129631448730622));
#33238=CARTESIAN_POINT('',(0.02115,-0.024,-0.0129631448730622));
#33239=CARTESIAN_POINT('',(0.02115,-0.008,-0.0129631448730622));
#33240=CARTESIAN_POINT('Origin',(0.01915000000001,-0.02400000000001,-0.0129631448730722));
#33241=CARTESIAN_POINT('Origin',(0.01915000000001,-0.00799999999999,-0.0129631448730722));
#33242=CARTESIAN_POINT('Origin',(0.02115,-0.016,0.0135625633639073));
#33243=CARTESIAN_POINT('',(0.02115,-0.008,0.0129631448730622));
#33244=CARTESIAN_POINT('',(0.02115,-0.024,0.0129631448730622));
#33245=CARTESIAN_POINT('',(0.0211500000000225,-0.008,0.0129631448730622));
#33246=CARTESIAN_POINT('',(0.02115000000001,-0.02400000000001,0.0135625633639173));
#33247=CARTESIAN_POINT('',(0.02115000000001,-0.00799999999999,0.0135625633639173));
#33248=CARTESIAN_POINT('Origin',(0.01915,-0.016,0.0129631448730622));
#33249=CARTESIAN_POINT('',(0.0208062162162162,-0.008,0.0140842817269487));
#33250=CARTESIAN_POINT('',(0.0208062162162162,-0.024,0.0140842817269487));
#33251=CARTESIAN_POINT('',(0.0208062162162262,-0.016,0.0140842817269587));
#33252=CARTESIAN_POINT('Origin',(0.01915000000001,-0.02400000000001,0.0129631448730722));
#33253=CARTESIAN_POINT('Origin',(0.01915000000001,-0.00799999999999,0.0129631448730722));
#33254=CARTESIAN_POINT('Origin',(-2.55351295663785E-17,-0.016,-3.88578058618804E-17));
#33255=CARTESIAN_POINT('',(0.0140842817269487,-0.024,0.0208062162162161));
#33256=CARTESIAN_POINT('',(0.0140842817269487,-0.008,0.0208062162162161));
#33257=CARTESIAN_POINT('',(0.0140842817269587,-0.016,0.0208062162162262));
#33258=CARTESIAN_POINT('Origin',(-1.00255351295664E-14,-0.02400000000001,
9.96114219413812E-15));
#33259=CARTESIAN_POINT('Origin',(-1.00255351295664E-14,-0.00799999999999,
9.96114219413812E-15));
#33260=CARTESIAN_POINT('Origin',(-0.01915,-0.016,-0.0129631448730623));
#33261=CARTESIAN_POINT('',(-0.0208062162162162,-0.008,-0.0140842817269487));
#33262=CARTESIAN_POINT('',(-0.0208062162162162,-0.024,-0.0140842817269487));
#33263=CARTESIAN_POINT('',(-0.0208062162162425,-0.008,-0.0140842817269665));
#33264=CARTESIAN_POINT('',(-0.02115,-0.024,-0.0129631448730623));
#33265=CARTESIAN_POINT('Origin',(-0.01915000000001,-0.02400000000001,-0.0129631448730723));
#33266=CARTESIAN_POINT('',(-0.02115,-0.008,-0.0129631448730623));
#33267=CARTESIAN_POINT('',(-0.0211500000000225,-0.008,-0.0129631448730623));
#33268=CARTESIAN_POINT('Origin',(-0.01915000000001,-0.00799999999999,-0.0129631448730723));
#33269=CARTESIAN_POINT('Origin',(-0.02115,-0.016,-0.0135625633639073));
#33270=CARTESIAN_POINT('',(-0.02115,-0.024,0.0129631448730623));
#33271=CARTESIAN_POINT('',(-0.02115000000001,-0.02400000000001,-0.0135625633639173));
#33272=CARTESIAN_POINT('',(-0.02115,-0.008,0.0129631448730623));
#33273=CARTESIAN_POINT('',(-0.02115,-0.008,0.0129631448730623));
#33274=CARTESIAN_POINT('',(-0.02115000000001,-0.00799999999999,-0.0135625633639173));
#33275=CARTESIAN_POINT('Origin',(-0.01915,-0.016,0.0129631448730623));
#33276=CARTESIAN_POINT('',(-0.0208062162162162,-0.024,0.0140842817269487));
#33277=CARTESIAN_POINT('Origin',(-0.01915000000001,-0.02400000000001,0.0129631448730723));
#33278=CARTESIAN_POINT('',(-0.0208062162162162,-0.008,0.0140842817269487));
#33279=CARTESIAN_POINT('',(-0.0208062162162381,-0.008,0.0140842817269635));
#33280=CARTESIAN_POINT('Origin',(-0.01915000000001,-0.00799999999999,0.0129631448730723));
#33281=CARTESIAN_POINT('Origin',(-2.55351295663785E-17,-0.016,-3.88578058618804E-17));
#33282=CARTESIAN_POINT('',(-0.0140842817269487,-0.024,0.0208062162162161));
#33283=CARTESIAN_POINT('Origin',(-1.00255351295664E-14,-0.02400000000001,
9.96114219413812E-15));
#33284=CARTESIAN_POINT('',(-0.0140842817269487,-0.008,0.0208062162162161));
#33285=CARTESIAN_POINT('',(-0.0140842817269643,-0.008,0.0208062162162391));
#33286=CARTESIAN_POINT('Origin',(-1.00255351295664E-14,-0.00799999999999,
9.96114219413812E-15));
#33287=CARTESIAN_POINT('Origin',(-0.0129631448730623,-0.016,0.01915));
#33288=CARTESIAN_POINT('',(-0.0129631448730623,-0.024,0.02115));
#33289=CARTESIAN_POINT('Origin',(-0.0129631448730723,-0.02400000000001,
0.01915000000001));
#33290=CARTESIAN_POINT('',(-0.0129631448730623,-0.008,0.02115));
#33291=CARTESIAN_POINT('',(-0.0129631448730623,-0.008,0.0211500000000225));
#33292=CARTESIAN_POINT('Origin',(-0.0129631448730723,-0.00799999999999,
0.01915000000001));
#33293=CARTESIAN_POINT('Origin',(-0.0135625633639073,-0.016,0.02115));
#33294=CARTESIAN_POINT('',(0.0129631448730622,-0.024,0.02115));
#33295=CARTESIAN_POINT('',(-0.0135625633639173,-0.02400000000001,0.0211500000000099));
#33296=CARTESIAN_POINT('',(0.0129631448730622,-0.008,0.02115));
#33297=CARTESIAN_POINT('',(0.0129631448730622,-0.008,0.02115));
#33298=CARTESIAN_POINT('',(-0.0135625633639173,-0.00799999999999,0.0211500000000099));
#33299=CARTESIAN_POINT('Origin',(0.0129631448730622,-0.016,0.01915));
#33300=CARTESIAN_POINT('Origin',(0.0129631448730722,-0.02400000000001,0.01915000000001));
#33301=CARTESIAN_POINT('Origin',(0.0129631448730722,-0.00799999999999,0.01915000000001));
#33302=CARTESIAN_POINT('Origin',(-1.4432899320127E-17,-0.024,-4.10782519111308E-17));
#33303=CARTESIAN_POINT('Origin',(-1.00255351295664E-14,-0.02400000000001,
9.96114219413812E-15));
#33304=CARTESIAN_POINT('',(0.0138,-0.02400000000001,0.0155));
#33305=CARTESIAN_POINT('Origin',(0.01550000000001,-0.02400000000001,0.01550000000001));
#33306=CARTESIAN_POINT('',(-0.0172,-0.02400000000001,-0.0155));
#33307=CARTESIAN_POINT('Origin',(-0.01550000000001,-0.02400000000001,-0.01550000000001));
#33308=CARTESIAN_POINT('',(0.0138,-0.02400000000001,-0.0155));
#33309=CARTESIAN_POINT('Origin',(0.01550000000001,-0.02400000000001,-0.01550000000001));
#33310=CARTESIAN_POINT('',(-0.0172,-0.02400000000001,0.0155));
#33311=CARTESIAN_POINT('Origin',(-0.01550000000001,-0.02400000000001,0.01550000000001));
#33312=CARTESIAN_POINT('',(-0.01915,-0.024,0.00793218971944474));
#33313=CARTESIAN_POINT('',(-0.0079321897194448,-0.024,0.01915));
#33314=CARTESIAN_POINT('',(-0.0079321897194548,-0.02400000000001,0.01915000000001));
#33315=CARTESIAN_POINT('',(0.00793218971944474,-0.024,0.01915));
#33316=CARTESIAN_POINT('',(0.00793218971945474,-0.02400000000001,0.01915000000001));
#33317=CARTESIAN_POINT('',(0.01915,-0.024,0.00793218971944472));
#33318=CARTESIAN_POINT('',(0.01915000000001,-0.02400000000001,0.00793218971945472));
#33319=CARTESIAN_POINT('',(0.01915,-0.024,-0.00793218971944482));
#33320=CARTESIAN_POINT('',(0.01915000000001,-0.02400000000001,-0.00793218971945483));
#33321=CARTESIAN_POINT('',(0.00793218971944474,-0.024,-0.01915));
#33322=CARTESIAN_POINT('',(0.00793218971945474,-0.02400000000001,-0.0191500000000101));
#33323=CARTESIAN_POINT('',(-0.00793218971944481,-0.024,-0.01915));
#33324=CARTESIAN_POINT('',(-0.00793218971945481,-0.02400000000001,-0.0191500000000101));
#33325=CARTESIAN_POINT('',(-0.01915,-0.024,-0.00793218971944481));
#33326=CARTESIAN_POINT('',(-0.01915000000001,-0.02400000000001,-0.00793218971945481));
#33327=CARTESIAN_POINT('',(-0.01915000000001,-0.02400000000001,0.00793218971945474));
#33328=CARTESIAN_POINT('Origin',(-2.55351295663785E-17,-0.016,-3.88578058618804E-17));
#33329=CARTESIAN_POINT('Origin',(-1.00255351295664E-14,-0.00799999999999,
9.96114219413812E-15));
#33330=CARTESIAN_POINT('Origin',(0.0155,-0.0699239856598395,0.0155));
#33331=CARTESIAN_POINT('',(0.0138,-0.00799999999999,0.0155));
#33332=CARTESIAN_POINT('',(0.0138,-0.0699239856598395,0.0155));
#33333=CARTESIAN_POINT('Origin',(0.01550000000001,-0.00799999999999,0.01550000000001));
#33334=CARTESIAN_POINT('Origin',(-0.0155,-0.0699239856598395,-0.0155));
#33335=CARTESIAN_POINT('',(-0.0172,-0.00799999999999,-0.0155));
#33336=CARTESIAN_POINT('',(-0.0172,-0.0699239856598395,-0.0155));
#33337=CARTESIAN_POINT('Origin',(-0.01550000000001,-0.00799999999999,-0.01550000000001));
#33338=CARTESIAN_POINT('Origin',(0.0155,-0.0699239856598395,-0.0155));
#33339=CARTESIAN_POINT('',(0.0138,-0.00799999999999,-0.0155));
#33340=CARTESIAN_POINT('',(0.0138,-0.0699239856598395,-0.0155));
#33341=CARTESIAN_POINT('Origin',(0.01550000000001,-0.00799999999999,-0.01550000000001));
#33342=CARTESIAN_POINT('Origin',(-0.0155,-0.0699239856598395,0.0155));
#33343=CARTESIAN_POINT('',(-0.0172,-0.00799999999999,0.0155));
#33344=CARTESIAN_POINT('',(-0.0172,-0.0699239856598395,0.0155));
#33345=CARTESIAN_POINT('Origin',(-0.01550000000001,-0.00799999999999,0.01550000000001));
#33346=CARTESIAN_POINT('Origin',(0.00793218971944474,-0.016,0.01915));
#33347=CARTESIAN_POINT('',(-0.0079321897194448,-0.008,0.01915));
#33348=CARTESIAN_POINT('',(-0.0079321897194548,-0.016,0.01915000000001));
#33349=CARTESIAN_POINT('',(0.00793218971944474,-0.008,0.01915));
#33350=CARTESIAN_POINT('',(0.00793218971945474,-0.00799999999999,0.01915000000001));
#33351=CARTESIAN_POINT('',(0.00793218971945474,-0.016,0.01915000000001));
#33352=CARTESIAN_POINT('Origin',(0.01915,-0.016,0.00793218971944472));
#33353=CARTESIAN_POINT('',(0.01915,-0.008,0.00793218971944472));
#33354=CARTESIAN_POINT('',(0.01915000000001,-0.00799999999999,0.00793218971945472));
#33355=CARTESIAN_POINT('',(0.01915000000001,-0.016,0.00793218971945472));
#33356=CARTESIAN_POINT('Origin',(0.01915,-0.016,-0.00793218971944482));
#33357=CARTESIAN_POINT('',(0.01915,-0.008,-0.00793218971944482));
#33358=CARTESIAN_POINT('',(0.01915000000001,-0.00799999999999,-0.00793218971945483));
#33359=CARTESIAN_POINT('',(0.01915000000001,-0.016,-0.00793218971945483));
#33360=CARTESIAN_POINT('Origin',(0.00793218971944474,-0.016,-0.01915));
#33361=CARTESIAN_POINT('',(0.00793218971944474,-0.008,-0.01915));
#33362=CARTESIAN_POINT('',(0.00793218971945474,-0.00799999999999,-0.0191500000000101));
#33363=CARTESIAN_POINT('',(0.00793218971945474,-0.016,-0.0191500000000101));
#33364=CARTESIAN_POINT('Origin',(-0.00793218971944481,-0.016,-0.01915));
#33365=CARTESIAN_POINT('',(-0.00793218971944481,-0.008,-0.01915));
#33366=CARTESIAN_POINT('',(-0.00793218971945481,-0.00799999999999,-0.0191500000000101));
#33367=CARTESIAN_POINT('',(-0.00793218971945481,-0.016,-0.0191500000000101));
#33368=CARTESIAN_POINT('Origin',(-0.01915,-0.016,-0.00793218971944481));
#33369=CARTESIAN_POINT('',(-0.01915,-0.008,-0.00793218971944481));
#33370=CARTESIAN_POINT('',(-0.01915000000001,-0.00799999999999,-0.00793218971945481));
#33371=CARTESIAN_POINT('',(-0.01915000000001,-0.016,-0.00793218971945481));
#33372=CARTESIAN_POINT('Origin',(-0.01915,-0.016,0.00793218971944474));
#33373=CARTESIAN_POINT('',(-0.01915,-0.008,0.00793218971944474));
#33374=CARTESIAN_POINT('',(-0.01915000000001,-0.00799999999999,0.00793218971945474));
#33375=CARTESIAN_POINT('',(-0.01915000000001,-0.016,0.00793218971945474));
#33376=CARTESIAN_POINT('Origin',(-0.0079321897194448,-0.016,0.01915));
#33377=CARTESIAN_POINT('',(-0.0079321897194548,-0.00799999999999,0.01915000000001));
#33378=CARTESIAN_POINT('Origin',(-1.4432899320127E-17,-0.008,-4.10782519111308E-17));
#34832=UNCERTAINTY_MEASURE_WITH_UNIT(LENGTH_MEASURE(1.E-5),#34877,
'DISTANCE_ACCURACY_VALUE',
'Maximum model space distance between geometric entities at asserted c
onnectivities');
#34841=UNCERTAINTY_MEASURE_WITH_UNIT(LENGTH_MEASURE(1.E-5),#34877,
'DISTANCE_ACCURACY_VALUE',
'Maximum model space distance between geometric entities at asserted c
onnectivities');
#34867=(
GEOMETRIC_REPRESENTATION_CONTEXT(3)
GLOBAL_UNCERTAINTY_ASSIGNED_CONTEXT((#34832))
GLOBAL_UNIT_ASSIGNED_CONTEXT((#34877,#34878,#34879))
REPRESENTATION_CONTEXT('','3D')
);
#34876=(
GEOMETRIC_REPRESENTATION_CONTEXT(3)
GLOBAL_UNCERTAINTY_ASSIGNED_CONTEXT((#34841))
GLOBAL_UNIT_ASSIGNED_CONTEXT((#34877,#34878,#34879))
REPRESENTATION_CONTEXT('','3D')
);
#34877=(
LENGTH_UNIT()
NAMED_UNIT(*)
SI_UNIT($,.METRE.)
);
#34878=(
NAMED_UNIT(*)
PLANE_ANGLE_UNIT()
SI_UNIT($,.RADIAN.)
);
#34879=(
NAMED_UNIT(*)
SI_UNIT($,.STERADIAN.)
SOLID_ANGLE_UNIT()
);
#34905=SHAPE_DEFINITION_REPRESENTATION(#34939,#35009);
#34939=PRODUCT_DEFINITION_SHAPE('',$,#35044);
#35009=SHAPE_REPRESENTATION('',(#21760),#34867);
#35018=PRODUCT_DEFINITION_CONTEXT('part definition',#35122,'design');
#35044=PRODUCT_DEFINITION('Motor Central Spacer','Motor Central Spacer',
#35078,#35018);
#35078=PRODUCT_DEFINITION_FORMATION('',$,#35149);
#35122=APPLICATION_CONTEXT('Managed model based 3d engineering');
#35123=PRODUCT_CONTEXT('part definition',#35122,'mechanical');
#35149=PRODUCT('Motor Central Spacer','Motor Central Spacer',
'LEGAL AND USAGE DISCLAIMER: this Data/Model is provided \X2\201C\X0\A
S IS\X2\201D\X0\ for informational and representational only. It is a 
geometric approximation and is NOT engineered, certified, or guarantee
d for dimensional accuracy, exact tolerances, or production-level prec
ision. Vendor disclaims all implied warranties including fitness for a
 particular purpose. DO NOT USE FOR DIRECT PHYSICAL MANUFACTURING, AUT
OMATED PRODUCTION, OR SAFETY-CRITICAL SYSTEMS without independent engi
neering verification and resolution of any design discrepancies.',(#35123));
#35166=PRESENTATION_STYLE_ASSIGNMENT((#35175));
#35175=SURFACE_STYLE_USAGE(.BOTH.,#35184);
#35184=SURFACE_SIDE_STYLE('',(#35193));
#35193=SURFACE_STYLE_FILL_AREA(#35202);
#35202=FILL_AREA_STYLE('Paint - Enamel Glossy (Grey)',(#35211));
#35211=FILL_AREA_STYLE_COLOUR('Paint - Enamel Glossy (Grey)',#35220);
#35220=COLOUR_RGB('Paint - Enamel Glossy (Grey)',0.701960784313725,0.701960784313725,
0.701960784313725);
ENDSEC;
END-ISO-10303-21;
